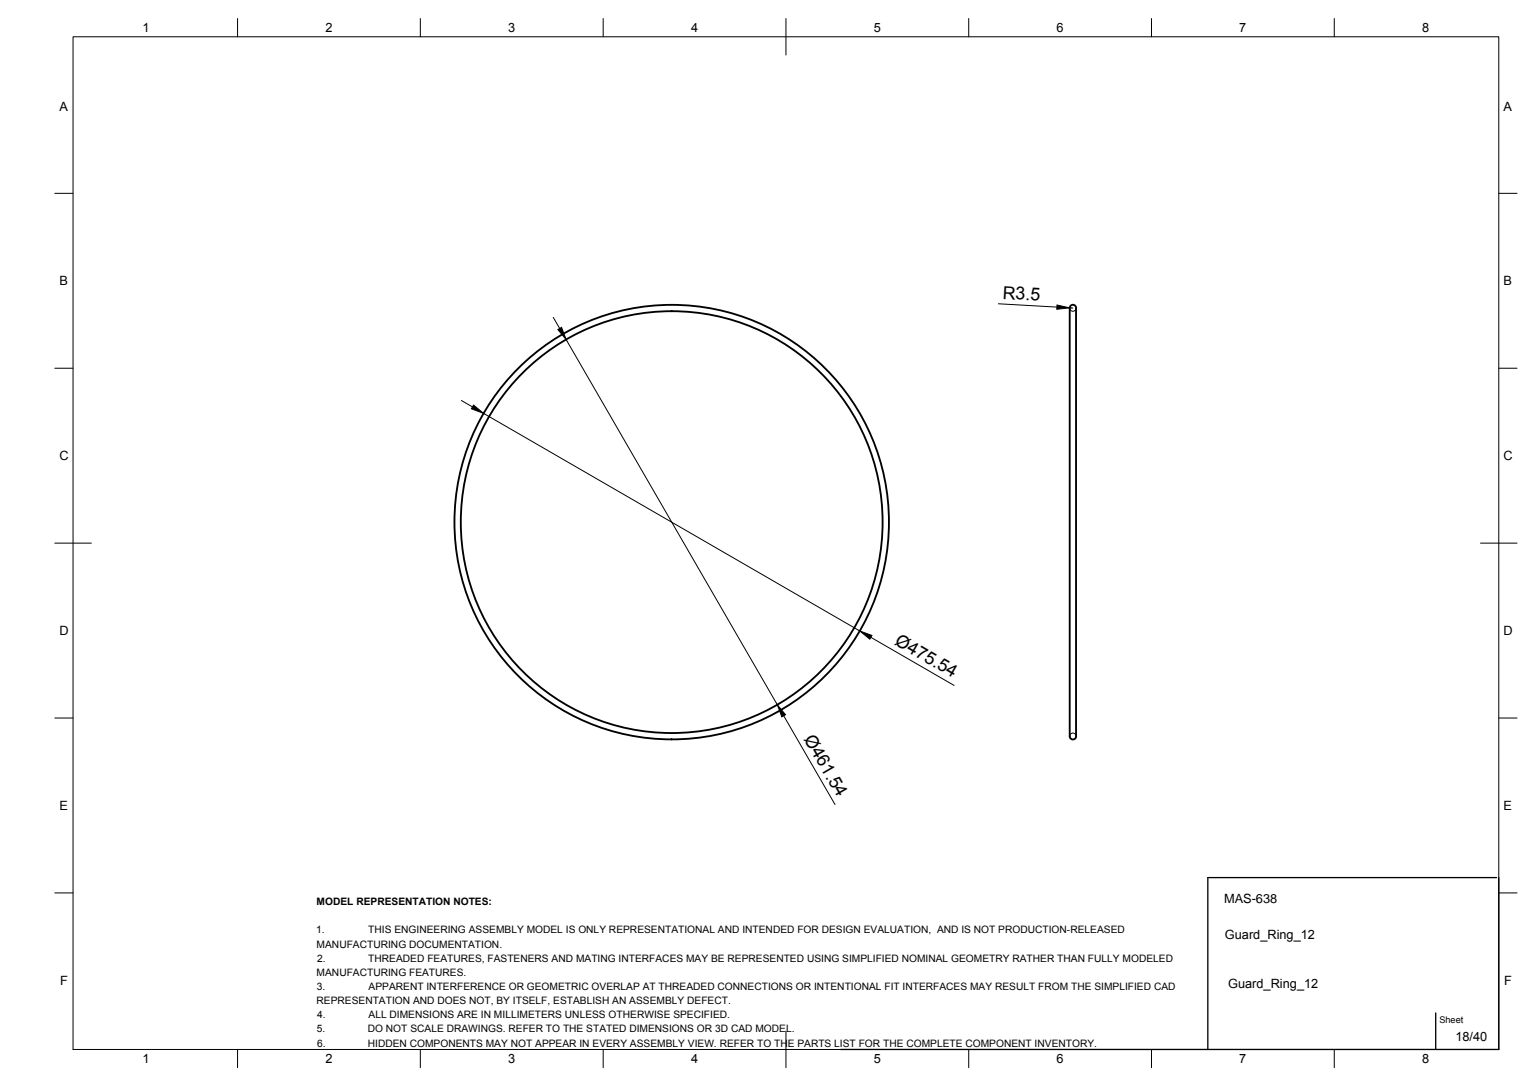
ISO-10303-21;
HEADER;
FILE_DESCRIPTION((''),'2;1');
FILE_NAME('Guard_Ring_12.step','2026-10-09T12:00:21-07:00',(''),(''),'','','');
FILE_SCHEMA (('AUTOMOTIVE_DESIGN { 1 0 10303 214 3 1 1 }'));
ENDSEC;
DATA;
#10=MECHANICAL_DESIGN_GEOMETRIC_PRESENTATION_REPRESENTATION('',(#413,#414),#10334);
#345=SHAPE_REPRESENTATION_RELATIONSHIP('SRR','None',#10461,#377) ;
#377=ADVANCED_BREP_SHAPE_REPRESENTATION('',(#449),#10313) ;
#413=STYLED_ITEM('',(#10631),#3378) ;
#414=STYLED_ITEM('',(#10632),#449) ;
#449=MANIFOLD_SOLID_BREP('Body1',#3571) ;
#870=FACE_OUTER_BOUND('',#1070,.T.) ;
#1070=EDGE_LOOP('',(#2393,#2394,#2395,#2396)) ;
#1298=CIRCLE('',#4019,0.349999999999999) ;
#1299=CIRCLE('',#4020,23.0768144613668) ;
#1524=VERTEX_POINT('',#5708) ;
#1853=EDGE_CURVE('',#1524,#1524,#1298,.T.) ;
#1854=EDGE_CURVE('',#1524,#1524,#1299,.T.) ;
#2393=ORIENTED_EDGE('',*,*,#1853,.F.) ;
#2394=ORIENTED_EDGE('',*,*,#1854,.T.) ;
#2395=ORIENTED_EDGE('',*,*,#1853,.T.) ;
#2396=ORIENTED_EDGE('',*,*,#1854,.F.) ;
#3316=TOROIDAL_SURFACE('',#4018,23.4268144613668,0.349999999999999) ;
#3378=ADVANCED_FACE('',(#870),#3316,.T.) ;
#3571=CLOSED_SHELL('',(#3378)) ;
#4017=AXIS2_PLACEMENT_3D('',#5706,#4595,#4596) ;
#4018=AXIS2_PLACEMENT_3D('',#5707,#4597,#4598) ;
#4019=AXIS2_PLACEMENT_3D('',#5709,#4599,#4600) ;
#4020=AXIS2_PLACEMENT_3D('',#5710,#4601,#4602) ;
#4595=DIRECTION('axis',(0.,0.,1.)) ;
#4596=DIRECTION('refdir',(1.,0.,0.)) ;
#4597=DIRECTION('center_axis',(-6.42891162084177E-17,-1.,-1.01883556321148E-16)) ;
#4598=DIRECTION('ref_axis',(1.,0.,0.)) ;
#4599=DIRECTION('center_axis',(0.,1.01883556321148E-16,-1.)) ;
#4600=DIRECTION('ref_axis',(-1.,0.,0.)) ;
#4601=DIRECTION('center_axis',(6.42891162084177E-17,1.,1.01883556321148E-16)) ;
#4602=DIRECTION('ref_axis',(1.,-6.42891162084177E-17,-6.55000379205715E-33)) ;
#5706=CARTESIAN_POINT('',(0.,0.,0.)) ;
#5707=CARTESIAN_POINT('Origin',(23.47768801576,67.3831179463143,68.2224337400009)) ;
#5708=CARTESIAN_POINT('',(0.400873554393198,67.3831179463143,68.2224337400009)) ;
#5709=CARTESIAN_POINT('Origin',(0.0508735543931991,67.3831179463143,68.2224337400009)) ;
#5710=CARTESIAN_POINT('Origin',(23.47768801576,67.3831179463143,68.2224337400009)) ;
#10276=UNCERTAINTY_MEASURE_WITH_UNIT(LENGTH_MEASURE(0.001),#10335,
'DISTANCE_ACCURACY_VALUE',
'Maximum model space distance between geometric entities at asserted c
onnectivities') ;
#10297=UNCERTAINTY_MEASURE_WITH_UNIT(LENGTH_MEASURE(0.001),#10335,
'DISTANCE_ACCURACY_VALUE',
'Maximum model space distance between geometric entities at asserted c
onnectivities') ;
#10313=(
GEOMETRIC_REPRESENTATION_CONTEXT(3)
GLOBAL_UNCERTAINTY_ASSIGNED_CONTEXT((#10276))
GLOBAL_UNIT_ASSIGNED_CONTEXT((#10335,#10337,#10338))
REPRESENTATION_CONTEXT('','3D')
) ;
#10334=(
GEOMETRIC_REPRESENTATION_CONTEXT(3)
GLOBAL_UNCERTAINTY_ASSIGNED_CONTEXT((#10297))
GLOBAL_UNIT_ASSIGNED_CONTEXT((#10335,#10337,#10338))
REPRESENTATION_CONTEXT('','3D')
) ;
#10335=(
LENGTH_UNIT()
NAMED_UNIT(*)
SI_UNIT(.CENTI.,.METRE.)
) ;
#10337=(
NAMED_UNIT(*)
PLANE_ANGLE_UNIT()
SI_UNIT($,.RADIAN.)
) ;
#10338=(
NAMED_UNIT(*)
SI_UNIT($,.STERADIAN.)
SOLID_ANGLE_UNIT()
) ;
#10354=SHAPE_DEFINITION_REPRESENTATION(#10390,#10461) ;
#10390=PRODUCT_DEFINITION_SHAPE('',$,#10498) ;
#10461=SHAPE_REPRESENTATION('',(#4017),#10313) ;
#10482=PRODUCT_DEFINITION_CONTEXT('part definition',#10592,'design') ;
#10498=PRODUCT_DEFINITION('Guard_Ring_12','Guard_Ring_12',#10534,#10482) ;
#10534=PRODUCT_DEFINITION_FORMATION('',$,#10609) ;
#10592=APPLICATION_CONTEXT(
'Core Data for Automotive Mechanical Design Process') ;
#10593=PRODUCT_CONTEXT('part definition',#10592,'mechanical') ;
#10609=PRODUCT('Guard_Ring_12','Guard_Ring_12',$,(#10593)) ;
#10631=PRESENTATION_STYLE_ASSIGNMENT((#10635)) ;
#10632=PRESENTATION_STYLE_ASSIGNMENT((#10636)) ;
#10635=SURFACE_STYLE_USAGE(.BOTH.,#10639) ;
#10636=SURFACE_STYLE_USAGE(.BOTH.,#10640) ;
#10639=SURFACE_SIDE_STYLE('',(#10643)) ;
#10640=SURFACE_SIDE_STYLE('',(#10644)) ;
#10643=SURFACE_STYLE_FILL_AREA(#10647) ;
#10644=SURFACE_STYLE_FILL_AREA(#10648) ;
#10647=FILL_AREA_STYLE('Opaque(25,25,25)',(#10651)) ;
#10648=FILL_AREA_STYLE('Opaque(202,209,238)',(#10652)) ;
#10651=FILL_AREA_STYLE_COLOUR('Opaque(25,25,25)',#10655) ;
#10652=FILL_AREA_STYLE_COLOUR('Opaque(202,209,238)',#10656) ;
#10655=COLOUR_RGB('Opaque(25,25,25)', 0.09019608, 0.27058824, 0.51372549) ;
#10656=COLOUR_RGB('Opaque(202,209,238)', 0.40784314, 0.44705882, 0.49803922) ;
ENDSEC;
END-ISO-10303-21;
